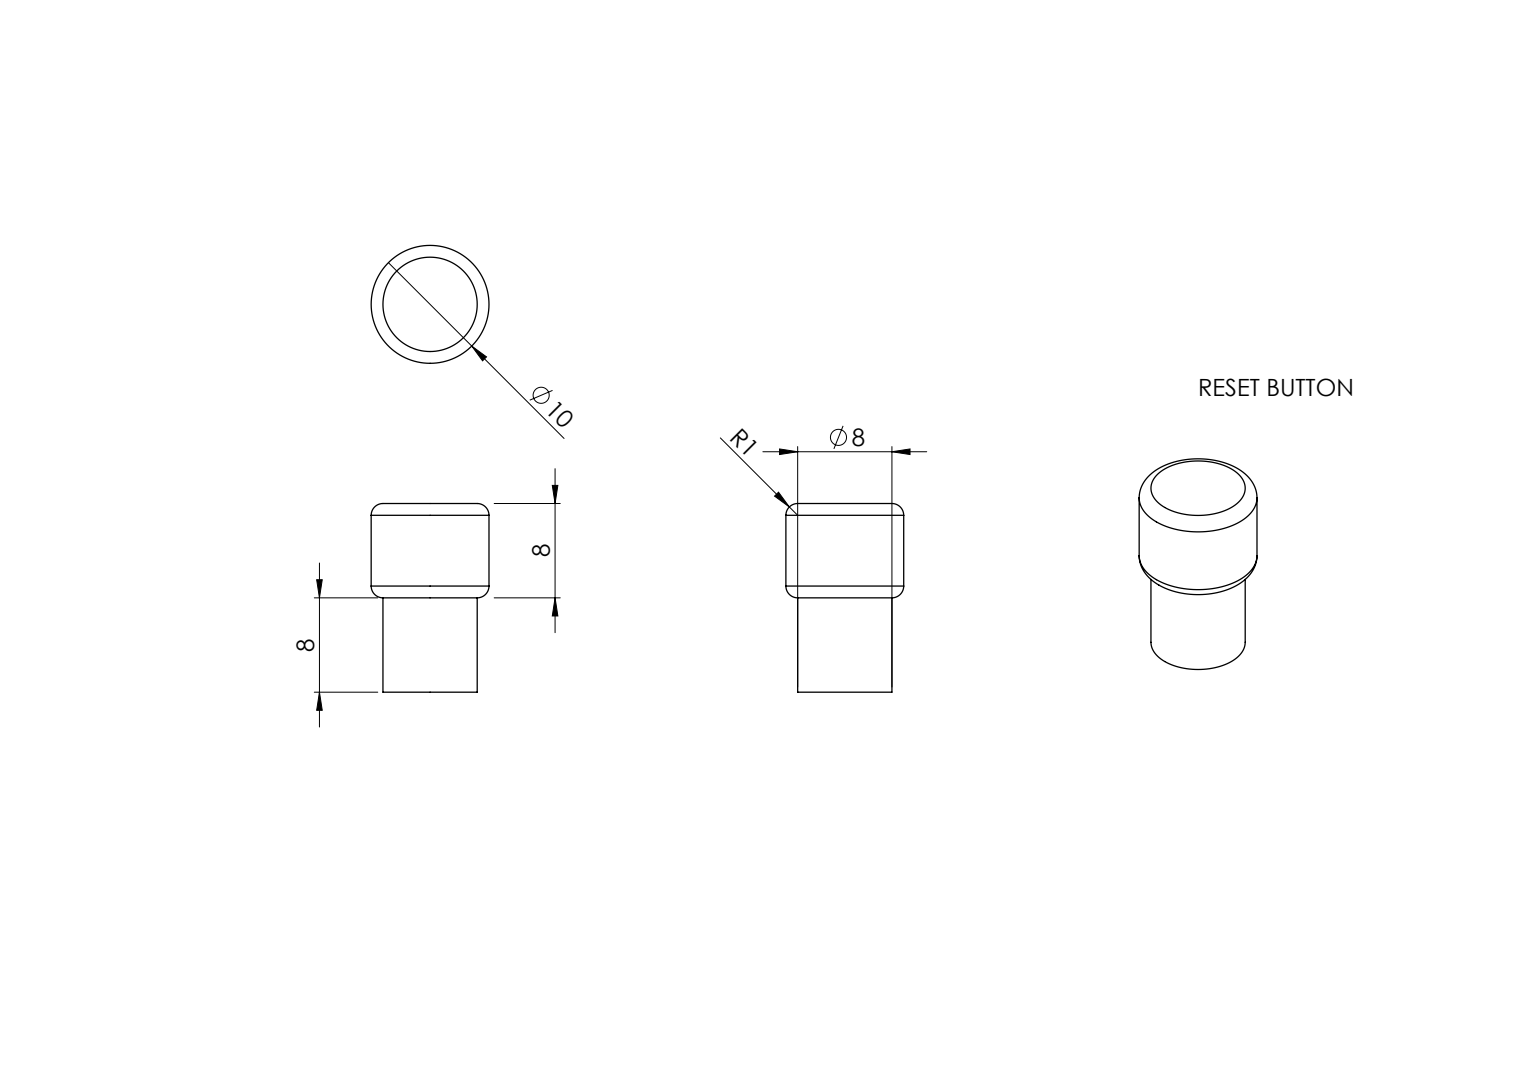
ISO-10303-21;
HEADER;
FILE_DESCRIPTION (('STEP AP214'),
    '1' );
FILE_NAME ('reset button.step',
    '2026-10-26T11:20:31',
    ( '' ),
    ( '' ),
    'SwSTEP 2.0',
    'SolidWorks 2026',
    '' );
FILE_SCHEMA (( 'AUTOMOTIVE_DESIGN' ));
ENDSEC;

DATA;
#10=MECHANICAL_DESIGN_GEOMETRIC_PRESENTATION_REPRESENTATION('',(#2667),#1914);
#71=EDGE_CURVE ( 'NONE', #1336, #2657, #200, .T. ) ;
#74=CARTESIAN_POINT ( 'NONE',  ( 3.469446951953614189E-15, 34.00000000000000000, 3.999999999999990674 ) ) ;
#90=AXIS2_PLACEMENT_3D ( 'NONE', #2223, #2270, #1567 ) ;
#91=EDGE_CURVE ( 'NONE', #668, #4199, #3027, .T. ) ;
#144=AXIS2_PLACEMENT_3D ( 'NONE', #3788, #1981, #1244 ) ;
#184=AXIS2_PLACEMENT_3D ( 'NONE', #568, #2063, #596 ) ;
#186=DIRECTION ( 'NONE',  ( 0.000000000000000000, 1.000000000000000000, 0.000000000000000000 ) ) ;
#200=LINE ( 'NONE', #2032, #3955 ) ;
#207=PRODUCT_DEFINITION_FORMATION_WITH_SPECIFIED_SOURCE ( 'ANY', '', #2064, .NOT_KNOWN. ) ;
#211=CARTESIAN_POINT ( 'NONE',  ( 3.469446951953614189E-15, 40.00000000000000000, 8.999999999999992895 ) ) ;
#235=CARTESIAN_POINT ( 'NONE',  ( 4.081770351527290718E-15, 41.00000000000000000, 13.99999999999999467 ) ) ;
#246=CARTESIAN_POINT ( 'NONE',  ( 3.469446951953614189E-15, 33.00000000000000000, 8.999999999999992895 ) ) ;
#263=( LENGTH_UNIT ( ) NAMED_UNIT ( * ) SI_UNIT ( .MILLI., .METRE. ) );
#270=DIRECTION ( 'NONE',  ( 0.000000000000000000, 0.000000000000000000, 1.000000000000000000 ) ) ;
#314=CARTESIAN_POINT ( 'NONE',  ( 3.469446951953614189E-15, 34.00000000000000000, 8.999999999999992895 ) ) ;
#325=DIRECTION ( 'NONE',  ( 0.000000000000000000, 0.000000000000000000, 1.000000000000000000 ) ) ;
#328=DIRECTION ( 'NONE',  ( 1.000000000000000000, -0.000000000000000000, 1.224646799147353207E-16 ) ) ;
#333=ORIENTED_EDGE ( 'NONE', *, *, #4326, .T. ) ;
#346=CARTESIAN_POINT ( 'NONE',  ( 3.469446951953614189E-15, 40.00000000000000000, 12.99999999999999467 ) ) ;
#349=CIRCLE ( 'NONE', #1112, 5.000000000000002665 ) ;
#381=FACE_OUTER_BOUND ( 'NONE', #4174, .T. ) ;
#387=AXIS2_PLACEMENT_3D ( 'NONE', #4457, #1221, #2661 ) ;
#410=EDGE_CURVE ( 'NONE', #1443, #3515, #349, .T. ) ;
#447=( LENGTH_UNIT ( ) NAMED_UNIT ( * ) SI_UNIT ( .MILLI., .METRE. ) );
#467=CIRCLE ( 'NONE', #1081, 1.000000000000000000 ) ;
#475=ORIENTED_EDGE ( 'NONE', *, *, #410, .F. ) ;
#491=FACE_OUTER_BOUND ( 'NONE', #3092, .T. ) ;
#520=AXIS2_PLACEMENT_3D ( 'NONE', #2929, #1829, #4028 ) ;
#526=ORIENTED_EDGE ( 'NONE', *, *, #71, .F. ) ;
#563=CARTESIAN_POINT ( 'NONE',  ( 4.020538011569923144E-15, 41.00000000000000000, 4.999999999999990230 ) ) ;
#568=CARTESIAN_POINT ( 'NONE',  ( 3.469446951953614189E-15, 37.00000000000000711, 8.999999999999992895 ) ) ;
#582=MECHANICAL_DESIGN_GEOMETRIC_PRESENTATION_REPRESENTATION('',(#2698),#3535);
#588=EDGE_LOOP ( 'NONE', ( #1122, #2733, #4479, #3461 ) ) ;
#590=APPLICATION_CONTEXT ( 'automotive_design' ) ;
#596=DIRECTION ( 'NONE',  ( 0.000000000000000000, 0.000000000000000000, -1.000000000000000000 ) ) ;
#600=ORIENTED_EDGE ( 'NONE', *, *, #1650, .T. ) ;
#622=ORIENTED_EDGE ( 'NONE', *, *, #410, .T. ) ;
#661=DIRECTION ( 'NONE',  ( 0.000000000000000000, 0.000000000000000000, 1.000000000000000000 ) ) ;
#663=AXIS2_PLACEMENT_3D ( 'NONE', #685, #3576, #3286 ) ;
#664=ADVANCED_FACE ( 'NONE', ( #491 ), #1842, .T. ) ;
#668=VERTEX_POINT ( 'NONE', #3651 ) ;
#680=AXIS2_PLACEMENT_3D ( 'NONE', #2681, #1906, #2998 ) ;
#685=CARTESIAN_POINT ( 'NONE',  ( 3.469446951953614189E-15, 33.00000000000000000, 8.999999999999992895 ) ) ;
#693=EDGE_CURVE ( 'NONE', #1443, #1195, #4565, .T. ) ;
#701=CARTESIAN_POINT ( 'NONE',  ( 3.959305671612554781E-15, 37.00000000000000711, 12.99999999999999289 ) ) ;
#718=CARTESIAN_POINT ( 'NONE',  ( 3.469446951953614189E-15, 41.00000000000000000, 8.999999999999992895 ) ) ;
#739=FILL_AREA_STYLE ('',( #3997 ) ) ;
#757=DIRECTION ( 'NONE',  ( 0.000000000000000000, 0.000000000000000000, -1.000000000000000000 ) ) ;
#784=ORIENTED_EDGE ( 'NONE', *, *, #2861, .T. ) ;
#808=VECTOR ( 'NONE', #923, 1000.000000000000000 ) ;
#821=CIRCLE ( 'NONE', #2478, 5.000000000000002665 ) ;
#826=EDGE_LOOP ( 'NONE', ( #4327, #1268 ) ) ;
#828=EDGE_CURVE ( 'NONE', #3515, #1443, #3541, .T. ) ;
#860=UNCERTAINTY_MEASURE_WITH_UNIT (LENGTH_MEASURE( 1.000000000000000082E-05 ), #447, 'distance_accuracy_value', 'NONE');
#864=EDGE_CURVE ( 'NONE', #668, #1336, #2102, .T. ) ;
#890=AXIS2_PLACEMENT_3D ( 'NONE', #718, #3932, #1027 ) ;
#894=DIRECTION ( 'NONE',  ( 0.000000000000000000, 1.000000000000000000, 0.000000000000000000 ) ) ;
#919=ORIENTED_EDGE ( 'NONE', *, *, #828, .T. ) ;
#921=AXIS2_PLACEMENT_3D ( 'NONE', #2968, #2293, #2676 ) ;
#923=DIRECTION ( 'NONE',  ( -0.000000000000000000, -1.000000000000000000, -0.000000000000000000 ) ) ;
#932=EDGE_CURVE ( 'NONE', #1142, #3862, #4379, .T. ) ;
#947=ORIENTED_EDGE ( 'NONE', *, *, #693, .T. ) ;
#989=CIRCLE ( 'NONE', #3032, 4.000000000000000000 ) ;
#1026=CIRCLE ( 'NONE', #2452, 4.000000000000000000 ) ;
#1027=DIRECTION ( 'NONE',  ( 0.000000000000000000, 0.000000000000000000, 1.000000000000000000 ) ) ;
#1081=AXIS2_PLACEMENT_3D ( 'NONE', #4311, #328, #1423 ) ;
#1099=ADVANCED_FACE ( 'NONE', ( #4046 ), #1518, .T. ) ;
#1112=AXIS2_PLACEMENT_3D ( 'NONE', #4369, #3581, #325 ) ;
#1122=ORIENTED_EDGE ( 'NONE', *, *, #1453, .F. ) ;
#1134=PRODUCT_CONTEXT ( 'NONE', #590, 'mechanical' ) ;
#1142=VERTEX_POINT ( 'NONE', #1213 ) ;
#1145=DIRECTION ( 'NONE',  ( 0.000000000000000000, 1.000000000000000000, 0.000000000000000000 ) ) ;
#1157=AXIS2_PLACEMENT_3D ( 'NONE', #3694, #1863, #2600 ) ;
#1188=SHAPE_REPRESENTATION_RELATIONSHIP ( 'NONE' , 'NONE' ,  #1892, #4552 ) ;
#1195=VERTEX_POINT ( 'NONE', #74 ) ;
#1211=ADVANCED_FACE ( 'NONE', ( #1238 ), #1489, .T. ) ;
#1213=CARTESIAN_POINT ( 'NONE',  ( 3.469446951953614189E-15, 41.00000000000000000, 12.99999999999999467 ) ) ;
#1216=ADVANCED_FACE ( 'NONE', ( #3782 ), #2633, .T. ) ;
#1221=DIRECTION ( 'NONE',  ( 0.000000000000000000, 1.000000000000000000, 0.000000000000000000 ) ) ;
#1238=FACE_OUTER_BOUND ( 'NONE', #2957, .T. ) ;
#1241=ORIENTED_EDGE ( 'NONE', *, *, #1971, .F. ) ;
#1244=DIRECTION ( 'NONE',  ( 0.000000000000000000, -0.000000000000000000, 1.000000000000000000 ) ) ;
#1263=LINE ( 'NONE', #235, #1850 ) ;
#1268=ORIENTED_EDGE ( 'NONE', *, *, #2581, .T. ) ;
#1272=( LENGTH_UNIT ( ) NAMED_UNIT ( * ) SI_UNIT ( .MILLI., .METRE. ) );
#1294=CIRCLE ( 'NONE', #3029, 1.000000000000000888 ) ;
#1316=CARTESIAN_POINT ( 'NONE',  ( 3.469446951953614189E-15, 34.00000000000000000, 12.99999999999999467 ) ) ;
#1329=MANIFOLD_SOLID_BREP ( 'Fillet1', #2747 ) ;
#1336=VERTEX_POINT ( 'NONE', #1689 ) ;
#1344=UNCERTAINTY_MEASURE_WITH_UNIT (LENGTH_MEASURE( 1.000000000000000082E-05 ), #1272, 'distance_accuracy_value', 'NONE');
#1379=( NAMED_UNIT ( * ) PLANE_ANGLE_UNIT ( ) SI_UNIT ( $, .RADIAN. ) );
#1413=AXIS2_PLACEMENT_3D ( 'NONE', #3396, #1582, #757 ) ;
#1423=DIRECTION ( 'NONE',  ( 1.224646799147350495E-16, 0.000000000000000000, -1.000000000000000000 ) ) ;
#1443=VERTEX_POINT ( 'NONE', #4697 ) ;
#1453=EDGE_CURVE ( 'NONE', #1443, #3862, #467, .T. ) ;
#1474=DIRECTION ( 'NONE',  ( -0.000000000000000000, -1.000000000000000000, -0.000000000000000000 ) ) ;
#1488=SURFACE_STYLE_FILL_AREA ( #739 ) ;
#1489=CYLINDRICAL_SURFACE ( 'NONE', #921, 5.000000000000001776 ) ;
#1491=EDGE_LOOP ( 'NONE', ( #4387, #919, #947, #2244 ) ) ;
#1509=VECTOR ( 'NONE', #4292, 1000.000000000000000 ) ;
#1518=TOROIDAL_SURFACE ( 'NONE', #90, 4.000000000000001776, 1.000000000000000000 ) ;
#1527=CIRCLE ( 'NONE', #2744, 4.000000000000000000 ) ;
#1547=DIRECTION ( 'NONE',  ( 0.000000000000000000, 0.000000000000000000, 1.000000000000000000 ) ) ;
#1555=PRODUCT_DEFINITION ( 'UNKNOWN', '', #207, #3519 ) ;
#1567=DIRECTION ( 'NONE',  ( 0.000000000000000000, 0.000000000000000000, 1.000000000000000000 ) ) ;
#1582=DIRECTION ( 'NONE',  ( -0.000000000000000000, -1.000000000000000000, -0.000000000000000000 ) ) ;
#1625=CARTESIAN_POINT ( 'NONE',  ( 3.959305671612554781E-15, 25.00000000000000000, 12.99999999999999289 ) ) ;
#1650=EDGE_CURVE ( 'NONE', #2657, #4199, #1527, .T. ) ;
#1656=DIRECTION ( 'NONE',  ( 0.000000000000000000, 0.000000000000000000, 1.000000000000000000 ) ) ;
#1666=AXIS2_PLACEMENT_3D ( 'NONE', #211, #186, #1656 ) ;
#1668=DIRECTION ( 'NONE',  ( -0.000000000000000000, -1.000000000000000000, -0.000000000000000000 ) ) ;
#1689=CARTESIAN_POINT ( 'NONE',  ( 3.469446951953614189E-15, 33.00000000000000000, 4.999999999999992006 ) ) ;
#1712=DIRECTION ( 'NONE',  ( 0.000000000000000000, 0.000000000000000000, 1.000000000000000000 ) ) ;
#1761=TOROIDAL_SURFACE ( 'NONE', #4422, 4.000000000000001776, 1.000000000000000000 ) ;
#1780=CARTESIAN_POINT ( 'NONE',  ( 0.000000000000000000, 0.000000000000000000, 0.000000000000000000 ) ) ;
#1807=CIRCLE ( 'NONE', #680, 4.000000000000001776 ) ;
#1824=SURFACE_SIDE_STYLE ('',( #1488 ) ) ;
#1828=EDGE_LOOP ( 'NONE', ( #3877, #4583, #4171, #2177 ) ) ;
#1829=DIRECTION ( 'NONE',  ( 0.000000000000000000, 1.000000000000000000, 0.000000000000000000 ) ) ;
#1842=CYLINDRICAL_SURFACE ( 'NONE', #1413, 4.000000000000000000 ) ;
#1850=VECTOR ( 'NONE', #4305, 1000.000000000000000 ) ;
#1863=DIRECTION ( 'NONE',  ( 1.000000000000000000, -0.000000000000000000, 1.224646799147353207E-16 ) ) ;
#1869=EDGE_CURVE ( 'NONE', #1336, #1195, #3133, .T. ) ;
#1880=FACE_OUTER_BOUND ( 'NONE', #4219, .T. ) ;
#1892=SHAPE_REPRESENTATION ( 'reset button', ( #2928 ), #4230 ) ;
#1906=DIRECTION ( 'NONE',  ( 0.000000000000000000, 1.000000000000000000, 0.000000000000000000 ) ) ;
#1912=EDGE_CURVE ( 'NONE', #3515, #1142, #4208, .T. ) ;
#1914=( GEOMETRIC_REPRESENTATION_CONTEXT ( 3 ) GLOBAL_UNCERTAINTY_ASSIGNED_CONTEXT ( ( #1344 ) ) GLOBAL_UNIT_ASSIGNED_CONTEXT ( ( #1272, #3758, #3450 ) ) REPRESENTATION_CONTEXT ( 'NONE', 'WORKASPACE' ) );
#1942=ADVANCED_FACE ( 'NONE', ( #381 ), #1761, .T. ) ;
#1951=SHAPE_DEFINITION_REPRESENTATION ( #2103, #1892 ) ;
#1970=CARTESIAN_POINT ( 'NONE',  ( 3.469446951953614189E-15, 41.00000000000000000, 3.999999999999990674 ) ) ;
#1971=EDGE_CURVE ( 'NONE', #1195, #3799, #2208, .T. ) ;
#1972=TOROIDAL_SURFACE ( 'NONE', #1666, 4.000000000000001776, 1.000000000000000000 ) ;
#1976=CARTESIAN_POINT ( 'NONE',  ( 3.469446951953614189E-15, 41.00000000000000000, 8.999999999999992895 ) ) ;
#1979=ORIENTED_EDGE ( 'NONE', *, *, #71, .T. ) ;
#1981=DIRECTION ( 'NONE',  ( 0.000000000000000000, 1.000000000000000000, 0.000000000000000000 ) ) ;
#1985=CARTESIAN_POINT ( 'NONE',  ( 3.469446951953614189E-15, 25.00000000000000000, 8.999999999999992895 ) ) ;
#1986=DIRECTION ( 'NONE',  ( 0.000000000000000000, 0.000000000000000000, 1.000000000000000000 ) ) ;
#1995=ORIENTED_EDGE ( 'NONE', *, *, #3041, .T. ) ;
#2032=CARTESIAN_POINT ( 'NONE',  ( 3.469446951953614189E-15, 37.00000000000000711, 4.999999999999992006 ) ) ;
#2063=DIRECTION ( 'NONE',  ( -0.000000000000000000, -1.000000000000000000, -0.000000000000000000 ) ) ;
#2064=PRODUCT ( 'reset button', 'reset button', '', ( #1134 ) ) ;
#2092=DIRECTION ( 'NONE',  ( 0.000000000000000000, 0.000000000000000000, 1.000000000000000000 ) ) ;
#2096=COLOUR_RGB ( '',0.8941176470588234615, 0.8941176470588234615, 0.8941176470588234615 ) ;
#2102=CIRCLE ( 'NONE', #663, 4.000000000000000000 ) ;
#2103=PRODUCT_DEFINITION_SHAPE ( 'NONE', 'NONE',  #1555 ) ;
#2134=ORIENTED_EDGE ( 'NONE', *, *, #4326, .F. ) ;
#2177=ORIENTED_EDGE ( 'NONE', *, *, #2861, .F. ) ;
#2208=CIRCLE ( 'NONE', #387, 5.000000000000002665 ) ;
#2223=CARTESIAN_POINT ( 'NONE',  ( 3.469446951953614189E-15, 40.00000000000000000, 8.999999999999992895 ) ) ;
#2244=ORIENTED_EDGE ( 'NONE', *, *, #1971, .T. ) ;
#2269=( NAMED_UNIT ( * ) PLANE_ANGLE_UNIT ( ) SI_UNIT ( $, .RADIAN. ) );
#2270=DIRECTION ( 'NONE',  ( 0.000000000000000000, 1.000000000000000000, 0.000000000000000000 ) ) ;
#2285=AXIS2_PLACEMENT_3D ( 'NONE', #346, #4344, #4367 ) ;
#2293=DIRECTION ( 'NONE',  ( -0.000000000000000000, -1.000000000000000000, -0.000000000000000000 ) ) ;
#2420=ADVANCED_FACE ( 'NONE', ( #4703 ), #3710, .T. ) ;
#2428=FACE_OUTER_BOUND ( 'NONE', #3876, .T. ) ;
#2452=AXIS2_PLACEMENT_3D ( 'NONE', #246, #894, #1986 ) ;
#2478=AXIS2_PLACEMENT_3D ( 'NONE', #314, #3936, #270 ) ;
#2496=CYLINDRICAL_SURFACE ( 'NONE', #3179, 5.000000000000001776 ) ;
#2529=( NAMED_UNIT ( * ) SI_UNIT ( $, .STERADIAN. ) SOLID_ANGLE_UNIT ( ) );
#2570=ADVANCED_FACE ( 'NONE', ( #1880 ), #3711, .F. ) ;
#2581=EDGE_CURVE ( 'NONE', #3862, #1142, #1807, .T. ) ;
#2600=DIRECTION ( 'NONE',  ( 1.224646799147350495E-16, 0.000000000000000000, -1.000000000000000000 ) ) ;
#2613=DIRECTION ( 'NONE',  ( 0.000000000000000000, 1.000000000000000000, 0.000000000000000000 ) ) ;
#2633=PLANE ( 'NONE',  #2738 ) ;
#2642=ORIENTED_EDGE ( 'NONE', *, *, #864, .F. ) ;
#2657=VERTEX_POINT ( 'NONE', #4481 ) ;
#2661=DIRECTION ( 'NONE',  ( 0.000000000000000000, 0.000000000000000000, 1.000000000000000000 ) ) ;
#2667=STYLED_ITEM('',(#4729),#1329);
#2676=DIRECTION ( 'NONE',  ( 0.000000000000000000, 0.000000000000000000, -1.000000000000000000 ) ) ;
#2681=CARTESIAN_POINT ( 'NONE',  ( 3.469446951953614189E-15, 41.00000000000000000, 8.999999999999992895 ) ) ;
#2698=STYLED_ITEM ( 'NONE', ( #4022 ), #4552 ) ;
#2728=CARTESIAN_POINT ( 'NONE',  ( 4.081770351527290718E-15, 40.00000000000000000, 13.99999999999999467 ) ) ;
#2733=ORIENTED_EDGE ( 'NONE', *, *, #828, .F. ) ;
#2738=AXIS2_PLACEMENT_3D ( 'NONE', #1976, #1145, #3323 ) ;
#2744=AXIS2_PLACEMENT_3D ( 'NONE', #3467, #3036, #3060 ) ;
#2747=CLOSED_SHELL ( 'NONE', ( #1099, #2420, #1211, #664, #3557, #2570, #3013, #1216, #1942, #3482 ) ) ;
#2861=EDGE_CURVE ( 'NONE', #668, #3799, #1294, .T. ) ;
#2928=AXIS2_PLACEMENT_3D ( 'NONE', #1780, #1712, #3957 ) ;
#2929=CARTESIAN_POINT ( 'NONE',  ( 3.469446951953614189E-15, 34.00000000000000000, 8.999999999999992895 ) ) ;
#2957=EDGE_LOOP ( 'NONE', ( #622, #3503, #4651, #4497 ) ) ;
#2968=CARTESIAN_POINT ( 'NONE',  ( 3.469446951953614189E-15, 41.00000000000000000, 8.999999999999992895 ) ) ;
#2988=ORIENTED_EDGE ( 'NONE', *, *, #91, .T. ) ;
#2998=DIRECTION ( 'NONE',  ( 0.000000000000000000, 0.000000000000000000, 1.000000000000000000 ) ) ;
#3011=CARTESIAN_POINT ( 'NONE',  ( 4.081770351527290718E-15, 34.00000000000000000, 13.99999999999999467 ) ) ;
#3013=ADVANCED_FACE ( 'NONE', ( #4434 ), #2496, .T. ) ;
#3027=LINE ( 'NONE', #701, #1509 ) ;
#3029=AXIS2_PLACEMENT_3D ( 'NONE', #1316, #4220, #2092 ) ;
#3032=AXIS2_PLACEMENT_3D ( 'NONE', #1985, #4132, #3842 ) ;
#3036=DIRECTION ( 'NONE',  ( 0.000000000000000000, 1.000000000000000000, 0.000000000000000000 ) ) ;
#3041=EDGE_CURVE ( 'NONE', #4199, #2657, #989, .T. ) ;
#3060=DIRECTION ( 'NONE',  ( 0.000000000000000000, 0.000000000000000000, 1.000000000000000000 ) ) ;
#3082=CARTESIAN_POINT ( 'NONE',  ( 3.469446951953614189E-15, 40.00000000000000000, 8.999999999999992895 ) ) ;
#3092=EDGE_LOOP ( 'NONE', ( #2642, #2988, #1995, #526 ) ) ;
#3099=ORIENTED_EDGE ( 'NONE', *, *, #1650, .F. ) ;
#3133=CIRCLE ( 'NONE', #1157, 1.000000000000000000 ) ;
#3146=EDGE_CURVE ( 'NONE', #3799, #1195, #821, .T. ) ;
#3179=AXIS2_PLACEMENT_3D ( 'NONE', #4010, #3264, #3241 ) ;
#3180=CYLINDRICAL_SURFACE ( 'NONE', #184, 4.000000000000000000 ) ;
#3230=( NAMED_UNIT ( * ) SI_UNIT ( $, .STERADIAN. ) SOLID_ANGLE_UNIT ( ) );
#3241=DIRECTION ( 'NONE',  ( 0.000000000000000000, 0.000000000000000000, -1.000000000000000000 ) ) ;
#3264=DIRECTION ( 'NONE',  ( -0.000000000000000000, -1.000000000000000000, -0.000000000000000000 ) ) ;
#3286=DIRECTION ( 'NONE',  ( 0.000000000000000000, 0.000000000000000000, 1.000000000000000000 ) ) ;
#3313=AXIS2_PLACEMENT_3D ( 'NONE', #3082, #1474, #661 ) ;
#3323=DIRECTION ( 'NONE',  ( 0.000000000000000000, -0.000000000000000000, 1.000000000000000000 ) ) ;
#3357=CARTESIAN_POINT ( 'NONE',  ( 3.469446951953614189E-15, 34.00000000000000000, 8.999999999999992895 ) ) ;
#3396=CARTESIAN_POINT ( 'NONE',  ( 3.469446951953614189E-15, 37.00000000000000711, 8.999999999999992895 ) ) ;
#3425=ORIENTED_EDGE ( 'NONE', *, *, #91, .F. ) ;
#3450=( NAMED_UNIT ( * ) SI_UNIT ( $, .STERADIAN. ) SOLID_ANGLE_UNIT ( ) );
#3461=ORIENTED_EDGE ( 'NONE', *, *, #2581, .F. ) ;
#3467=CARTESIAN_POINT ( 'NONE',  ( 3.469446951953614189E-15, 25.00000000000000000, 8.999999999999992895 ) ) ;
#3482=ADVANCED_FACE ( 'NONE', ( #3533 ), #1972, .T. ) ;
#3503=ORIENTED_EDGE ( 'NONE', *, *, #3577, .T. ) ;
#3515=VERTEX_POINT ( 'NONE', #2728 ) ;
#3519=PRODUCT_DEFINITION_CONTEXT ( 'detailed design', #3836, 'design' ) ;
#3533=FACE_OUTER_BOUND ( 'NONE', #588, .T. ) ;
#3535=( GEOMETRIC_REPRESENTATION_CONTEXT ( 3 ) GLOBAL_UNCERTAINTY_ASSIGNED_CONTEXT ( ( #860 ) ) GLOBAL_UNIT_ASSIGNED_CONTEXT ( ( #447, #2269, #2529 ) ) REPRESENTATION_CONTEXT ( 'NONE', 'WORKASPACE' ) );
#3541=CIRCLE ( 'NONE', #3313, 5.000000000000002665 ) ;
#3557=ADVANCED_FACE ( 'NONE', ( #2428 ), #3180, .T. ) ;
#3576=DIRECTION ( 'NONE',  ( 0.000000000000000000, 1.000000000000000000, 0.000000000000000000 ) ) ;
#3577=EDGE_CURVE ( 'NONE', #3515, #3799, #1263, .T. ) ;
#3581=DIRECTION ( 'NONE',  ( -0.000000000000000000, -1.000000000000000000, -0.000000000000000000 ) ) ;
#3635=ORIENTED_EDGE ( 'NONE', *, *, #1453, .T. ) ;
#3651=CARTESIAN_POINT ( 'NONE',  ( 3.959305671612554781E-15, 33.00000000000000000, 12.99999999999999289 ) ) ;
#3659=ORIENTED_EDGE ( 'NONE', *, *, #3041, .F. ) ;
#3694=CARTESIAN_POINT ( 'NONE',  ( 3.959305671612555570E-15, 34.00000000000000000, 4.999999999999990230 ) ) ;
#3710=TOROIDAL_SURFACE ( 'NONE', #520, 4.000000000000001776, 1.000000000000000000 ) ;
#3711=PLANE ( 'NONE',  #144 ) ;
#3758=( NAMED_UNIT ( * ) PLANE_ANGLE_UNIT ( ) SI_UNIT ( $, .RADIAN. ) );
#3782=FACE_OUTER_BOUND ( 'NONE', #826, .T. ) ;
#3788=CARTESIAN_POINT ( 'NONE',  ( 3.469446951953614189E-15, 25.00000000000000000, 8.999999999999992895 ) ) ;
#3799=VERTEX_POINT ( 'NONE', #3011 ) ;
#3836=APPLICATION_CONTEXT ( 'automotive_design' ) ;
#3842=DIRECTION ( 'NONE',  ( 0.000000000000000000, 0.000000000000000000, 1.000000000000000000 ) ) ;
#3862=VERTEX_POINT ( 'NONE', #563 ) ;
#3876=EDGE_LOOP ( 'NONE', ( #3425, #2134, #1979, #600 ) ) ;
#3877=ORIENTED_EDGE ( 'NONE', *, *, #864, .T. ) ;
#3932=DIRECTION ( 'NONE',  ( 0.000000000000000000, 1.000000000000000000, 0.000000000000000000 ) ) ;
#3936=DIRECTION ( 'NONE',  ( 0.000000000000000000, 1.000000000000000000, 0.000000000000000000 ) ) ;
#3955=VECTOR ( 'NONE', #1668, 1000.000000000000000 ) ;
#3957=DIRECTION ( 'NONE',  ( 1.000000000000000000, 0.000000000000000000, 0.000000000000000000 ) ) ;
#3997=FILL_AREA_STYLE_COLOUR ( '', #2096 ) ;
#4010=CARTESIAN_POINT ( 'NONE',  ( 3.469446951953614189E-15, 41.00000000000000000, 8.999999999999992895 ) ) ;
#4022=PRESENTATION_STYLE_ASSIGNMENT (( #4449 ) ) ;
#4025=ORIENTED_EDGE ( 'NONE', *, *, #1869, .F. ) ;
#4028=DIRECTION ( 'NONE',  ( 0.000000000000000000, 0.000000000000000000, 1.000000000000000000 ) ) ;
#4046=FACE_OUTER_BOUND ( 'NONE', #4499, .T. ) ;
#4132=DIRECTION ( 'NONE',  ( 0.000000000000000000, 1.000000000000000000, 0.000000000000000000 ) ) ;
#4150=UNCERTAINTY_MEASURE_WITH_UNIT (LENGTH_MEASURE( 1.000000000000000082E-05 ), #263, 'distance_accuracy_value', 'NONE');
#4171=ORIENTED_EDGE ( 'NONE', *, *, #3146, .F. ) ;
#4174=EDGE_LOOP ( 'NONE', ( #4025, #333, #784, #1241 ) ) ;
#4199=VERTEX_POINT ( 'NONE', #1625 ) ;
#4208=CIRCLE ( 'NONE', #2285, 1.000000000000000888 ) ;
#4219=EDGE_LOOP ( 'NONE', ( #3099, #3659 ) ) ;
#4220=DIRECTION ( 'NONE',  ( -1.000000000000000000, 0.000000000000000000, 0.000000000000000000 ) ) ;
#4230=( GEOMETRIC_REPRESENTATION_CONTEXT ( 3 ) GLOBAL_UNCERTAINTY_ASSIGNED_CONTEXT ( ( #4150 ) ) GLOBAL_UNIT_ASSIGNED_CONTEXT ( ( #263, #1379, #3230 ) ) REPRESENTATION_CONTEXT ( 'NONE', 'WORKASPACE' ) );
#4292=DIRECTION ( 'NONE',  ( -0.000000000000000000, -1.000000000000000000, -0.000000000000000000 ) ) ;
#4305=DIRECTION ( 'NONE',  ( -0.000000000000000000, -1.000000000000000000, -0.000000000000000000 ) ) ;
#4311=CARTESIAN_POINT ( 'NONE',  ( 3.959305671612555570E-15, 40.00000000000000000, 4.999999999999990230 ) ) ;
#4326=EDGE_CURVE ( 'NONE', #1336, #668, #1026, .T. ) ;
#4327=ORIENTED_EDGE ( 'NONE', *, *, #932, .T. ) ;
#4344=DIRECTION ( 'NONE',  ( -1.000000000000000000, 0.000000000000000000, 0.000000000000000000 ) ) ;
#4357=ORIENTED_EDGE ( 'NONE', *, *, #1912, .F. ) ;
#4367=DIRECTION ( 'NONE',  ( 0.000000000000000000, 0.000000000000000000, 1.000000000000000000 ) ) ;
#4369=CARTESIAN_POINT ( 'NONE',  ( 3.469446951953614189E-15, 40.00000000000000000, 8.999999999999992895 ) ) ;
#4379=CIRCLE ( 'NONE', #890, 4.000000000000001776 ) ;
#4387=ORIENTED_EDGE ( 'NONE', *, *, #3577, .F. ) ;
#4422=AXIS2_PLACEMENT_3D ( 'NONE', #3357, #2613, #1547 ) ;
#4434=FACE_OUTER_BOUND ( 'NONE', #1491, .T. ) ;
#4449=SURFACE_STYLE_USAGE ( .BOTH. , #1824 ) ;
#4457=CARTESIAN_POINT ( 'NONE',  ( 3.469446951953614189E-15, 34.00000000000000000, 8.999999999999992895 ) ) ;
#4479=ORIENTED_EDGE ( 'NONE', *, *, #1912, .T. ) ;
#4481=CARTESIAN_POINT ( 'NONE',  ( 3.469446951953614189E-15, 25.00000000000000000, 4.999999999999992006 ) ) ;
#4497=ORIENTED_EDGE ( 'NONE', *, *, #693, .F. ) ;
#4499=EDGE_LOOP ( 'NONE', ( #475, #3635, #4694, #4357 ) ) ;
#4552=ADVANCED_BREP_SHAPE_REPRESENTATION ( '', ( #1329, #2928 ), #4230 ) ;
#4565=LINE ( 'NONE', #1970, #808 ) ;
#4583=ORIENTED_EDGE ( 'NONE', *, *, #1869, .T. ) ;
#4651=ORIENTED_EDGE ( 'NONE', *, *, #3146, .T. ) ;
#4694=ORIENTED_EDGE ( 'NONE', *, *, #932, .F. ) ;
#4697=CARTESIAN_POINT ( 'NONE',  ( 3.469446951953614189E-15, 40.00000000000000000, 3.999999999999990674 ) ) ;
#4703=FACE_OUTER_BOUND ( 'NONE', #1828, .T. ) ;
#4723=COLOUR_RGB('Light Blue',0.38,0.62,0.78);
#4724=FILL_AREA_STYLE_COLOUR('',#4723);
#4725=FILL_AREA_STYLE('',(#4724));
#4726=SURFACE_STYLE_FILL_AREA(#4725);
#4727=SURFACE_SIDE_STYLE('',(#4726));
#4728=SURFACE_STYLE_USAGE(.BOTH.,#4727);
#4729=PRESENTATION_STYLE_ASSIGNMENT((#4728));
ENDSEC;
END-ISO-10303-21;
